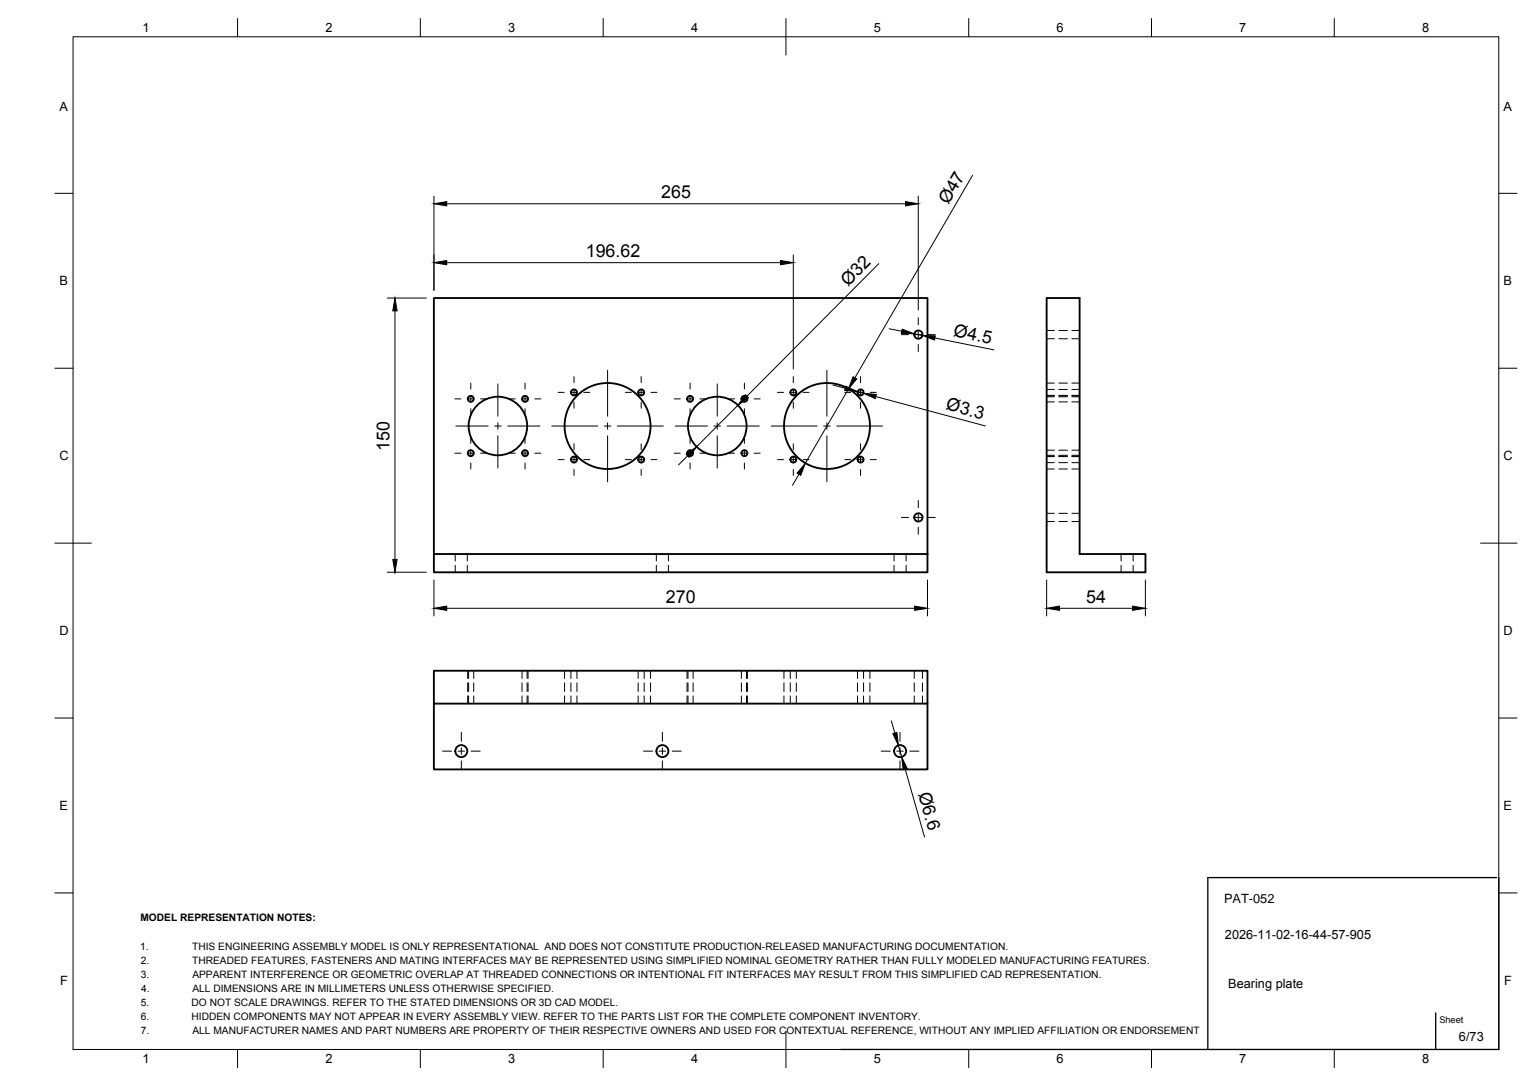
ISO-10303-21;
HEADER;
/* Generated by software containing ST-Developer
 * from STEP Tools, Inc. (www.steptools.com) 
 */

FILE_DESCRIPTION(
/* description */ ('Hand-crank gear train demonstrator'),
/* implementation_level */ '2;1');

FILE_NAME(
/* name */ 'Bearing plate.step',
/* time_stamp */ '2026-10-28T03:22:13-07:00',
/* author */ (''),
/* organization */ (''),
/* preprocessor_version */ 'ST-DEVELOPER v20.2',
/* originating_system */ 'Autodesk Translation Framework v15.17.0.0',
/* authorisation */ '');

FILE_SCHEMA (('AUTOMOTIVE_DESIGN { 1 0 10303 214 3 1 1 }'));
ENDSEC;

DATA;
#10=MECHANICAL_DESIGN_GEOMETRIC_PRESENTATION_REPRESENTATION('',(#1190),#62758);
#1062=SHAPE_REPRESENTATION_RELATIONSHIP('SRR','None',#63034,#1126);
#1126=ADVANCED_BREP_SHAPE_REPRESENTATION('',(#1269),#62688);
#1190=STYLED_ITEM('',(#63462),#1269);
#1269=MANIFOLD_SOLID_BREP('Body1',#16370);
#1348=FACE_BOUND('',#3100,.T.);
#1349=FACE_BOUND('',#3101,.T.);
#1350=FACE_BOUND('',#3102,.T.);
#1351=FACE_BOUND('',#3105,.T.);
#1352=FACE_BOUND('',#3106,.T.);
#1353=FACE_BOUND('',#3107,.T.);
#1354=FACE_BOUND('',#3108,.T.);
#1355=FACE_BOUND('',#3109,.T.);
#1356=FACE_BOUND('',#3110,.T.);
#1357=FACE_BOUND('',#3111,.T.);
#1358=FACE_BOUND('',#3112,.T.);
#1359=FACE_BOUND('',#3113,.T.);
#1360=FACE_BOUND('',#3114,.T.);
#1361=FACE_BOUND('',#3115,.T.);
#1362=FACE_BOUND('',#3116,.T.);
#1363=FACE_BOUND('',#3117,.T.);
#1364=FACE_BOUND('',#3118,.T.);
#1365=FACE_BOUND('',#3119,.T.);
#1366=FACE_BOUND('',#3120,.T.);
#1367=FACE_BOUND('',#3121,.T.);
#1368=FACE_BOUND('',#3122,.T.);
#1369=FACE_BOUND('',#3123,.T.);
#1370=FACE_BOUND('',#3124,.T.);
#1371=FACE_BOUND('',#3125,.T.);
#1372=FACE_BOUND('',#3126,.T.);
#1373=FACE_BOUND('',#3129,.T.);
#1374=FACE_BOUND('',#3130,.T.);
#1375=FACE_BOUND('',#3131,.T.);
#1376=FACE_BOUND('',#3132,.T.);
#1377=FACE_BOUND('',#3133,.T.);
#1378=FACE_BOUND('',#3134,.T.);
#1379=FACE_BOUND('',#3135,.T.);
#1380=FACE_BOUND('',#3136,.T.);
#1381=FACE_BOUND('',#3137,.T.);
#1382=FACE_BOUND('',#3138,.T.);
#1383=FACE_BOUND('',#3139,.T.);
#1384=FACE_BOUND('',#3140,.T.);
#1385=FACE_BOUND('',#3141,.T.);
#1386=FACE_BOUND('',#3142,.T.);
#1387=FACE_BOUND('',#3143,.T.);
#1388=FACE_BOUND('',#3144,.T.);
#1389=FACE_BOUND('',#3145,.T.);
#1390=FACE_BOUND('',#3146,.T.);
#1391=FACE_BOUND('',#3147,.T.);
#1392=FACE_BOUND('',#3148,.T.);
#1393=FACE_BOUND('',#3149,.T.);
#1394=FACE_BOUND('',#3150,.T.);
#1395=FACE_BOUND('',#3154,.T.);
#1396=FACE_BOUND('',#3155,.T.);
#1397=FACE_BOUND('',#3156,.T.);
#1639=PLANE('',#17252);
#1640=PLANE('',#17253);
#1641=PLANE('',#17254);
#1642=PLANE('',#17255);
#1643=PLANE('',#17256);
#1644=PLANE('',#17257);
#1645=PLANE('',#17258);
#1646=PLANE('',#17259);
#2132=FACE_OUTER_BOUND('',#3074,.T.);
#2133=FACE_OUTER_BOUND('',#3075,.T.);
#2134=FACE_OUTER_BOUND('',#3076,.T.);
#2135=FACE_OUTER_BOUND('',#3077,.T.);
#2136=FACE_OUTER_BOUND('',#3078,.T.);
#2137=FACE_OUTER_BOUND('',#3079,.T.);
#2138=FACE_OUTER_BOUND('',#3080,.T.);
#2139=FACE_OUTER_BOUND('',#3081,.T.);
#2140=FACE_OUTER_BOUND('',#3082,.T.);
#2141=FACE_OUTER_BOUND('',#3083,.T.);
#2142=FACE_OUTER_BOUND('',#3084,.T.);
#2143=FACE_OUTER_BOUND('',#3085,.T.);
#2144=FACE_OUTER_BOUND('',#3086,.T.);
#2145=FACE_OUTER_BOUND('',#3087,.T.);
#2146=FACE_OUTER_BOUND('',#3088,.T.);
#2147=FACE_OUTER_BOUND('',#3089,.T.);
#2148=FACE_OUTER_BOUND('',#3090,.T.);
#2149=FACE_OUTER_BOUND('',#3091,.T.);
#2150=FACE_OUTER_BOUND('',#3092,.T.);
#2151=FACE_OUTER_BOUND('',#3093,.T.);
#2152=FACE_OUTER_BOUND('',#3094,.T.);
#2153=FACE_OUTER_BOUND('',#3095,.T.);
#2154=FACE_OUTER_BOUND('',#3096,.T.);
#2155=FACE_OUTER_BOUND('',#3097,.T.);
#2156=FACE_OUTER_BOUND('',#3098,.T.);
#2157=FACE_OUTER_BOUND('',#3099,.T.);
#2158=FACE_OUTER_BOUND('',#3103,.T.);
#2159=FACE_OUTER_BOUND('',#3104,.T.);
#2160=FACE_OUTER_BOUND('',#3127,.T.);
#2161=FACE_OUTER_BOUND('',#3128,.T.);
#2162=FACE_OUTER_BOUND('',#3151,.T.);
#2163=FACE_OUTER_BOUND('',#3152,.T.);
#2164=FACE_OUTER_BOUND('',#3153,.T.);
#3074=EDGE_LOOP('',(#10877,#10878,#10879,#10880));
#3075=EDGE_LOOP('',(#10881,#10882,#10883,#10884));
#3076=EDGE_LOOP('',(#10885,#10886,#10887,#10888));
#3077=EDGE_LOOP('',(#10889,#10890,#10891,#10892));
#3078=EDGE_LOOP('',(#10893,#10894,#10895,#10896));
#3079=EDGE_LOOP('',(#10897,#10898,#10899,#10900));
#3080=EDGE_LOOP('',(#10901,#10902,#10903,#10904));
#3081=EDGE_LOOP('',(#10905,#10906,#10907,#10908));
#3082=EDGE_LOOP('',(#10909,#10910,#10911,#10912));
#3083=EDGE_LOOP('',(#10913,#10914,#10915,#10916));
#3084=EDGE_LOOP('',(#10917,#10918,#10919,#10920));
#3085=EDGE_LOOP('',(#10921,#10922,#10923,#10924));
#3086=EDGE_LOOP('',(#10925,#10926,#10927,#10928));
#3087=EDGE_LOOP('',(#10929,#10930,#10931,#10932));
#3088=EDGE_LOOP('',(#10933,#10934,#10935,#10936));
#3089=EDGE_LOOP('',(#10937,#10938,#10939,#10940));
#3090=EDGE_LOOP('',(#10941,#10942,#10943,#10944));
#3091=EDGE_LOOP('',(#10945,#10946,#10947,#10948));
#3092=EDGE_LOOP('',(#10949,#10950,#10951,#10952));
#3093=EDGE_LOOP('',(#10953,#10954,#10955,#10956));
#3094=EDGE_LOOP('',(#10957,#10958,#10959,#10960));
#3095=EDGE_LOOP('',(#10961,#10962,#10963,#10964));
#3096=EDGE_LOOP('',(#10965,#10966,#10967,#10968));
#3097=EDGE_LOOP('',(#10969,#10970,#10971,#10972));
#3098=EDGE_LOOP('',(#10973,#10974,#10975,#10976));
#3099=EDGE_LOOP('',(#10977,#10978,#10979,#10980));
#3100=EDGE_LOOP('',(#10981));
#3101=EDGE_LOOP('',(#10982));
#3102=EDGE_LOOP('',(#10983));
#3103=EDGE_LOOP('',(#10984,#10985,#10986,#10987));
#3104=EDGE_LOOP('',(#10988,#10989,#10990,#10991));
#3105=EDGE_LOOP('',(#10992));
#3106=EDGE_LOOP('',(#10993));
#3107=EDGE_LOOP('',(#10994));
#3108=EDGE_LOOP('',(#10995));
#3109=EDGE_LOOP('',(#10996));
#3110=EDGE_LOOP('',(#10997));
#3111=EDGE_LOOP('',(#10998));
#3112=EDGE_LOOP('',(#10999));
#3113=EDGE_LOOP('',(#11000));
#3114=EDGE_LOOP('',(#11001));
#3115=EDGE_LOOP('',(#11002));
#3116=EDGE_LOOP('',(#11003));
#3117=EDGE_LOOP('',(#11004));
#3118=EDGE_LOOP('',(#11005));
#3119=EDGE_LOOP('',(#11006));
#3120=EDGE_LOOP('',(#11007));
#3121=EDGE_LOOP('',(#11008));
#3122=EDGE_LOOP('',(#11009));
#3123=EDGE_LOOP('',(#11010));
#3124=EDGE_LOOP('',(#11011));
#3125=EDGE_LOOP('',(#11012));
#3126=EDGE_LOOP('',(#11013));
#3127=EDGE_LOOP('',(#11014,#11015,#11016,#11017,#11018,#11019));
#3128=EDGE_LOOP('',(#11020,#11021,#11022,#11023));
#3129=EDGE_LOOP('',(#11024));
#3130=EDGE_LOOP('',(#11025));
#3131=EDGE_LOOP('',(#11026));
#3132=EDGE_LOOP('',(#11027));
#3133=EDGE_LOOP('',(#11028));
#3134=EDGE_LOOP('',(#11029));
#3135=EDGE_LOOP('',(#11030));
#3136=EDGE_LOOP('',(#11031));
#3137=EDGE_LOOP('',(#11032));
#3138=EDGE_LOOP('',(#11033));
#3139=EDGE_LOOP('',(#11034));
#3140=EDGE_LOOP('',(#11035));
#3141=EDGE_LOOP('',(#11036));
#3142=EDGE_LOOP('',(#11037));
#3143=EDGE_LOOP('',(#11038));
#3144=EDGE_LOOP('',(#11039));
#3145=EDGE_LOOP('',(#11040));
#3146=EDGE_LOOP('',(#11041));
#3147=EDGE_LOOP('',(#11042));
#3148=EDGE_LOOP('',(#11043));
#3149=EDGE_LOOP('',(#11044));
#3150=EDGE_LOOP('',(#11045));
#3151=EDGE_LOOP('',(#11046,#11047,#11048,#11049,#11050,#11051));
#3152=EDGE_LOOP('',(#11052,#11053,#11054,#11055));
#3153=EDGE_LOOP('',(#11056,#11057,#11058,#11059));
#3154=EDGE_LOOP('',(#11060));
#3155=EDGE_LOOP('',(#11061));
#3156=EDGE_LOOP('',(#11062));
#4301=LINE('',#23361,#5433);
#4302=LINE('',#23367,#5434);
#4303=LINE('',#23373,#5435);
#4304=LINE('',#23379,#5436);
#4305=LINE('',#23385,#5437);
#4306=LINE('',#23391,#5438);
#4307=LINE('',#23397,#5439);
#4308=LINE('',#23403,#5440);
#4309=LINE('',#23409,#5441);
#4310=LINE('',#23415,#5442);
#4311=LINE('',#23421,#5443);
#4312=LINE('',#23427,#5444);
#4313=LINE('',#23433,#5445);
#4314=LINE('',#23439,#5446);
#4315=LINE('',#23445,#5447);
#4316=LINE('',#23451,#5448);
#4317=LINE('',#23457,#5449);
#4318=LINE('',#23463,#5450);
#4319=LINE('',#23469,#5451);
#4320=LINE('',#23475,#5452);
#4321=LINE('',#23481,#5453);
#4322=LINE('',#23487,#5454);
#4323=LINE('',#23493,#5455);
#4324=LINE('',#23499,#5456);
#4325=LINE('',#23505,#5457);
#4326=LINE('',#23510,#5458);
#4327=LINE('',#23512,#5459);
#4328=LINE('',#23514,#5460);
#4329=LINE('',#23515,#5461);
#4330=LINE('',#23518,#5462);
#4331=LINE('',#23520,#5463);
#4332=LINE('',#23521,#5464);
#4333=LINE('',#23525,#5465);
#4334=LINE('',#23527,#5466);
#4335=LINE('',#23529,#5467);
#4336=LINE('',#23530,#5468);
#4337=LINE('',#23532,#5469);
#4338=LINE('',#23534,#5470);
#4339=LINE('',#23535,#5471);
#4340=LINE('',#23538,#5472);
#4341=LINE('',#23539,#5473);
#4342=LINE('',#23541,#5474);
#4343=LINE('',#23542,#5475);
#5433=VECTOR('',#18888,0.225000000000001);
#5434=VECTOR('',#18895,0.225000000000001);
#5435=VECTOR('',#18902,0.164999999999999);
#5436=VECTOR('',#18909,0.164999999999999);
#5437=VECTOR('',#18916,0.164999999999999);
#5438=VECTOR('',#18923,0.164999999999999);
#5439=VECTOR('',#18930,2.35);
#5440=VECTOR('',#18937,0.164999999999999);
#5441=VECTOR('',#18944,0.164999999999999);
#5442=VECTOR('',#18951,0.164999999999999);
#5443=VECTOR('',#18958,0.164999999999999);
#5444=VECTOR('',#18965,1.6);
#5445=VECTOR('',#18972,0.165);
#5446=VECTOR('',#18979,0.165);
#5447=VECTOR('',#18986,0.165);
#5448=VECTOR('',#18993,0.165);
#5449=VECTOR('',#19000,2.35);
#5450=VECTOR('',#19007,0.165);
#5451=VECTOR('',#19014,0.165);
#5452=VECTOR('',#19021,0.165);
#5453=VECTOR('',#19028,0.165);
#5454=VECTOR('',#19035,1.6);
#5455=VECTOR('',#19042,0.33);
#5456=VECTOR('',#19049,0.33);
#5457=VECTOR('',#19056,0.329999999999998);
#5458=VECTOR('',#19061,1.);
#5459=VECTOR('',#19062,1.);
#5460=VECTOR('',#19063,1.);
#5461=VECTOR('',#19064,1.);
#5462=VECTOR('',#19067,1.);
#5463=VECTOR('',#19068,1.);
#5464=VECTOR('',#19069,1.);
#5465=VECTOR('',#19072,1.);
#5466=VECTOR('',#19073,1.);
#5467=VECTOR('',#19074,1.);
#5468=VECTOR('',#19075,1.);
#5469=VECTOR('',#19078,1.);
#5470=VECTOR('',#19079,1.);
#5471=VECTOR('',#19080,1.);
#5472=VECTOR('',#19083,1.);
#5473=VECTOR('',#19084,1.);
#5474=VECTOR('',#19087,1.);
#5475=VECTOR('',#19088,1.);
#6556=CIRCLE('',#17178,0.225000000000001);
#6557=CIRCLE('',#17179,0.225000000000001);
#6558=CIRCLE('',#17181,0.225000000000001);
#6559=CIRCLE('',#17182,0.225000000000001);
#6560=CIRCLE('',#17184,0.164999999999999);
#6561=CIRCLE('',#17185,0.164999999999999);
#6562=CIRCLE('',#17187,0.164999999999999);
#6563=CIRCLE('',#17188,0.164999999999999);
#6564=CIRCLE('',#17190,0.164999999999999);
#6565=CIRCLE('',#17191,0.164999999999999);
#6566=CIRCLE('',#17193,0.164999999999999);
#6567=CIRCLE('',#17194,0.164999999999999);
#6568=CIRCLE('',#17196,2.35);
#6569=CIRCLE('',#17197,2.35);
#6570=CIRCLE('',#17199,0.164999999999999);
#6571=CIRCLE('',#17200,0.164999999999999);
#6572=CIRCLE('',#17202,0.164999999999999);
#6573=CIRCLE('',#17203,0.164999999999999);
#6574=CIRCLE('',#17205,0.164999999999999);
#6575=CIRCLE('',#17206,0.164999999999999);
#6576=CIRCLE('',#17208,0.164999999999999);
#6577=CIRCLE('',#17209,0.164999999999999);
#6578=CIRCLE('',#17211,1.6);
#6579=CIRCLE('',#17212,1.6);
#6580=CIRCLE('',#17214,0.165);
#6581=CIRCLE('',#17215,0.165);
#6582=CIRCLE('',#17217,0.165);
#6583=CIRCLE('',#17218,0.165);
#6584=CIRCLE('',#17220,0.165);
#6585=CIRCLE('',#17221,0.165);
#6586=CIRCLE('',#17223,0.165);
#6587=CIRCLE('',#17224,0.165);
#6588=CIRCLE('',#17226,2.35);
#6589=CIRCLE('',#17227,2.35);
#6590=CIRCLE('',#17229,0.165);
#6591=CIRCLE('',#17230,0.165);
#6592=CIRCLE('',#17232,0.165);
#6593=CIRCLE('',#17233,0.165);
#6594=CIRCLE('',#17235,0.165);
#6595=CIRCLE('',#17236,0.165);
#6596=CIRCLE('',#17238,0.165);
#6597=CIRCLE('',#17239,0.165);
#6598=CIRCLE('',#17241,1.6);
#6599=CIRCLE('',#17242,1.6);
#6600=CIRCLE('',#17244,0.33);
#6601=CIRCLE('',#17245,0.33);
#6602=CIRCLE('',#17247,0.33);
#6603=CIRCLE('',#17248,0.33);
#6604=CIRCLE('',#17250,0.329999999999998);
#6605=CIRCLE('',#17251,0.329999999999998);
#7226=VERTEX_POINT('',#23358);
#7227=VERTEX_POINT('',#23360);
#7228=VERTEX_POINT('',#23364);
#7229=VERTEX_POINT('',#23366);
#7230=VERTEX_POINT('',#23370);
#7231=VERTEX_POINT('',#23372);
#7232=VERTEX_POINT('',#23376);
#7233=VERTEX_POINT('',#23378);
#7234=VERTEX_POINT('',#23382);
#7235=VERTEX_POINT('',#23384);
#7236=VERTEX_POINT('',#23388);
#7237=VERTEX_POINT('',#23390);
#7238=VERTEX_POINT('',#23394);
#7239=VERTEX_POINT('',#23396);
#7240=VERTEX_POINT('',#23400);
#7241=VERTEX_POINT('',#23402);
#7242=VERTEX_POINT('',#23406);
#7243=VERTEX_POINT('',#23408);
#7244=VERTEX_POINT('',#23412);
#7245=VERTEX_POINT('',#23414);
#7246=VERTEX_POINT('',#23418);
#7247=VERTEX_POINT('',#23420);
#7248=VERTEX_POINT('',#23424);
#7249=VERTEX_POINT('',#23426);
#7250=VERTEX_POINT('',#23430);
#7251=VERTEX_POINT('',#23432);
#7252=VERTEX_POINT('',#23436);
#7253=VERTEX_POINT('',#23438);
#7254=VERTEX_POINT('',#23442);
#7255=VERTEX_POINT('',#23444);
#7256=VERTEX_POINT('',#23448);
#7257=VERTEX_POINT('',#23450);
#7258=VERTEX_POINT('',#23454);
#7259=VERTEX_POINT('',#23456);
#7260=VERTEX_POINT('',#23460);
#7261=VERTEX_POINT('',#23462);
#7262=VERTEX_POINT('',#23466);
#7263=VERTEX_POINT('',#23468);
#7264=VERTEX_POINT('',#23472);
#7265=VERTEX_POINT('',#23474);
#7266=VERTEX_POINT('',#23478);
#7267=VERTEX_POINT('',#23480);
#7268=VERTEX_POINT('',#23484);
#7269=VERTEX_POINT('',#23486);
#7270=VERTEX_POINT('',#23490);
#7271=VERTEX_POINT('',#23492);
#7272=VERTEX_POINT('',#23496);
#7273=VERTEX_POINT('',#23498);
#7274=VERTEX_POINT('',#23502);
#7275=VERTEX_POINT('',#23504);
#7276=VERTEX_POINT('',#23508);
#7277=VERTEX_POINT('',#23509);
#7278=VERTEX_POINT('',#23511);
#7279=VERTEX_POINT('',#23513);
#7280=VERTEX_POINT('',#23517);
#7281=VERTEX_POINT('',#23519);
#7282=VERTEX_POINT('',#23523);
#7283=VERTEX_POINT('',#23524);
#7284=VERTEX_POINT('',#23526);
#7285=VERTEX_POINT('',#23528);
#7286=VERTEX_POINT('',#23533);
#7287=VERTEX_POINT('',#23537);
#8690=EDGE_CURVE('',#7226,#7226,#6556,.T.);
#8691=EDGE_CURVE('',#7226,#7227,#4301,.T.);
#8692=EDGE_CURVE('',#7227,#7227,#6557,.T.);
#8693=EDGE_CURVE('',#7228,#7228,#6558,.T.);
#8694=EDGE_CURVE('',#7228,#7229,#4302,.T.);
#8695=EDGE_CURVE('',#7229,#7229,#6559,.T.);
#8696=EDGE_CURVE('',#7230,#7230,#6560,.T.);
#8697=EDGE_CURVE('',#7230,#7231,#4303,.T.);
#8698=EDGE_CURVE('',#7231,#7231,#6561,.T.);
#8699=EDGE_CURVE('',#7232,#7232,#6562,.T.);
#8700=EDGE_CURVE('',#7232,#7233,#4304,.T.);
#8701=EDGE_CURVE('',#7233,#7233,#6563,.T.);
#8702=EDGE_CURVE('',#7234,#7234,#6564,.T.);
#8703=EDGE_CURVE('',#7234,#7235,#4305,.T.);
#8704=EDGE_CURVE('',#7235,#7235,#6565,.T.);
#8705=EDGE_CURVE('',#7236,#7236,#6566,.T.);
#8706=EDGE_CURVE('',#7236,#7237,#4306,.T.);
#8707=EDGE_CURVE('',#7237,#7237,#6567,.T.);
#8708=EDGE_CURVE('',#7238,#7238,#6568,.T.);
#8709=EDGE_CURVE('',#7238,#7239,#4307,.T.);
#8710=EDGE_CURVE('',#7239,#7239,#6569,.T.);
#8711=EDGE_CURVE('',#7240,#7240,#6570,.T.);
#8712=EDGE_CURVE('',#7240,#7241,#4308,.T.);
#8713=EDGE_CURVE('',#7241,#7241,#6571,.T.);
#8714=EDGE_CURVE('',#7242,#7242,#6572,.T.);
#8715=EDGE_CURVE('',#7242,#7243,#4309,.T.);
#8716=EDGE_CURVE('',#7243,#7243,#6573,.T.);
#8717=EDGE_CURVE('',#7244,#7244,#6574,.T.);
#8718=EDGE_CURVE('',#7244,#7245,#4310,.T.);
#8719=EDGE_CURVE('',#7245,#7245,#6575,.T.);
#8720=EDGE_CURVE('',#7246,#7246,#6576,.T.);
#8721=EDGE_CURVE('',#7246,#7247,#4311,.T.);
#8722=EDGE_CURVE('',#7247,#7247,#6577,.T.);
#8723=EDGE_CURVE('',#7248,#7248,#6578,.T.);
#8724=EDGE_CURVE('',#7248,#7249,#4312,.T.);
#8725=EDGE_CURVE('',#7249,#7249,#6579,.T.);
#8726=EDGE_CURVE('',#7250,#7250,#6580,.T.);
#8727=EDGE_CURVE('',#7250,#7251,#4313,.T.);
#8728=EDGE_CURVE('',#7251,#7251,#6581,.T.);
#8729=EDGE_CURVE('',#7252,#7252,#6582,.T.);
#8730=EDGE_CURVE('',#7252,#7253,#4314,.T.);
#8731=EDGE_CURVE('',#7253,#7253,#6583,.T.);
#8732=EDGE_CURVE('',#7254,#7254,#6584,.T.);
#8733=EDGE_CURVE('',#7254,#7255,#4315,.T.);
#8734=EDGE_CURVE('',#7255,#7255,#6585,.T.);
#8735=EDGE_CURVE('',#7256,#7256,#6586,.T.);
#8736=EDGE_CURVE('',#7256,#7257,#4316,.T.);
#8737=EDGE_CURVE('',#7257,#7257,#6587,.T.);
#8738=EDGE_CURVE('',#7258,#7258,#6588,.T.);
#8739=EDGE_CURVE('',#7258,#7259,#4317,.T.);
#8740=EDGE_CURVE('',#7259,#7259,#6589,.T.);
#8741=EDGE_CURVE('',#7260,#7260,#6590,.T.);
#8742=EDGE_CURVE('',#7260,#7261,#4318,.T.);
#8743=EDGE_CURVE('',#7261,#7261,#6591,.T.);
#8744=EDGE_CURVE('',#7262,#7262,#6592,.T.);
#8745=EDGE_CURVE('',#7262,#7263,#4319,.T.);
#8746=EDGE_CURVE('',#7263,#7263,#6593,.T.);
#8747=EDGE_CURVE('',#7264,#7264,#6594,.T.);
#8748=EDGE_CURVE('',#7264,#7265,#4320,.T.);
#8749=EDGE_CURVE('',#7265,#7265,#6595,.T.);
#8750=EDGE_CURVE('',#7266,#7266,#6596,.T.);
#8751=EDGE_CURVE('',#7266,#7267,#4321,.T.);
#8752=EDGE_CURVE('',#7267,#7267,#6597,.T.);
#8753=EDGE_CURVE('',#7268,#7268,#6598,.T.);
#8754=EDGE_CURVE('',#7268,#7269,#4322,.T.);
#8755=EDGE_CURVE('',#7269,#7269,#6599,.T.);
#8756=EDGE_CURVE('',#7270,#7270,#6600,.T.);
#8757=EDGE_CURVE('',#7270,#7271,#4323,.T.);
#8758=EDGE_CURVE('',#7271,#7271,#6601,.T.);
#8759=EDGE_CURVE('',#7272,#7272,#6602,.T.);
#8760=EDGE_CURVE('',#7272,#7273,#4324,.T.);
#8761=EDGE_CURVE('',#7273,#7273,#6603,.T.);
#8762=EDGE_CURVE('',#7274,#7274,#6604,.T.);
#8763=EDGE_CURVE('',#7274,#7275,#4325,.T.);
#8764=EDGE_CURVE('',#7275,#7275,#6605,.T.);
#8765=EDGE_CURVE('',#7276,#7277,#4326,.T.);
#8766=EDGE_CURVE('',#7276,#7278,#4327,.T.);
#8767=EDGE_CURVE('',#7279,#7278,#4328,.T.);
#8768=EDGE_CURVE('',#7277,#7279,#4329,.T.);
#8769=EDGE_CURVE('',#7277,#7280,#4330,.T.);
#8770=EDGE_CURVE('',#7280,#7281,#4331,.T.);
#8771=EDGE_CURVE('',#7281,#7276,#4332,.T.);
#8772=EDGE_CURVE('',#7282,#7283,#4333,.T.);
#8773=EDGE_CURVE('',#7283,#7284,#4334,.T.);
#8774=EDGE_CURVE('',#7285,#7284,#4335,.T.);
#8775=EDGE_CURVE('',#7282,#7285,#4336,.T.);
#8776=EDGE_CURVE('',#7281,#7282,#4337,.T.);
#8777=EDGE_CURVE('',#7286,#7285,#4338,.T.);
#8778=EDGE_CURVE('',#7278,#7286,#4339,.T.);
#8779=EDGE_CURVE('',#7287,#7286,#4340,.T.);
#8780=EDGE_CURVE('',#7279,#7287,#4341,.T.);
#8781=EDGE_CURVE('',#7283,#7280,#4342,.T.);
#8782=EDGE_CURVE('',#7284,#7287,#4343,.T.);
#10877=ORIENTED_EDGE('',*,*,#8690,.F.);
#10878=ORIENTED_EDGE('',*,*,#8691,.T.);
#10879=ORIENTED_EDGE('',*,*,#8692,.F.);
#10880=ORIENTED_EDGE('',*,*,#8691,.F.);
#10881=ORIENTED_EDGE('',*,*,#8693,.F.);
#10882=ORIENTED_EDGE('',*,*,#8694,.T.);
#10883=ORIENTED_EDGE('',*,*,#8695,.F.);
#10884=ORIENTED_EDGE('',*,*,#8694,.F.);
#10885=ORIENTED_EDGE('',*,*,#8696,.F.);
#10886=ORIENTED_EDGE('',*,*,#8697,.T.);
#10887=ORIENTED_EDGE('',*,*,#8698,.F.);
#10888=ORIENTED_EDGE('',*,*,#8697,.F.);
#10889=ORIENTED_EDGE('',*,*,#8699,.F.);
#10890=ORIENTED_EDGE('',*,*,#8700,.T.);
#10891=ORIENTED_EDGE('',*,*,#8701,.F.);
#10892=ORIENTED_EDGE('',*,*,#8700,.F.);
#10893=ORIENTED_EDGE('',*,*,#8702,.F.);
#10894=ORIENTED_EDGE('',*,*,#8703,.T.);
#10895=ORIENTED_EDGE('',*,*,#8704,.F.);
#10896=ORIENTED_EDGE('',*,*,#8703,.F.);
#10897=ORIENTED_EDGE('',*,*,#8705,.F.);
#10898=ORIENTED_EDGE('',*,*,#8706,.T.);
#10899=ORIENTED_EDGE('',*,*,#8707,.F.);
#10900=ORIENTED_EDGE('',*,*,#8706,.F.);
#10901=ORIENTED_EDGE('',*,*,#8708,.F.);
#10902=ORIENTED_EDGE('',*,*,#8709,.T.);
#10903=ORIENTED_EDGE('',*,*,#8710,.F.);
#10904=ORIENTED_EDGE('',*,*,#8709,.F.);
#10905=ORIENTED_EDGE('',*,*,#8711,.F.);
#10906=ORIENTED_EDGE('',*,*,#8712,.T.);
#10907=ORIENTED_EDGE('',*,*,#8713,.F.);
#10908=ORIENTED_EDGE('',*,*,#8712,.F.);
#10909=ORIENTED_EDGE('',*,*,#8714,.F.);
#10910=ORIENTED_EDGE('',*,*,#8715,.T.);
#10911=ORIENTED_EDGE('',*,*,#8716,.F.);
#10912=ORIENTED_EDGE('',*,*,#8715,.F.);
#10913=ORIENTED_EDGE('',*,*,#8717,.F.);
#10914=ORIENTED_EDGE('',*,*,#8718,.T.);
#10915=ORIENTED_EDGE('',*,*,#8719,.F.);
#10916=ORIENTED_EDGE('',*,*,#8718,.F.);
#10917=ORIENTED_EDGE('',*,*,#8720,.F.);
#10918=ORIENTED_EDGE('',*,*,#8721,.T.);
#10919=ORIENTED_EDGE('',*,*,#8722,.F.);
#10920=ORIENTED_EDGE('',*,*,#8721,.F.);
#10921=ORIENTED_EDGE('',*,*,#8723,.F.);
#10922=ORIENTED_EDGE('',*,*,#8724,.T.);
#10923=ORIENTED_EDGE('',*,*,#8725,.F.);
#10924=ORIENTED_EDGE('',*,*,#8724,.F.);
#10925=ORIENTED_EDGE('',*,*,#8726,.F.);
#10926=ORIENTED_EDGE('',*,*,#8727,.T.);
#10927=ORIENTED_EDGE('',*,*,#8728,.F.);
#10928=ORIENTED_EDGE('',*,*,#8727,.F.);
#10929=ORIENTED_EDGE('',*,*,#8729,.F.);
#10930=ORIENTED_EDGE('',*,*,#8730,.T.);
#10931=ORIENTED_EDGE('',*,*,#8731,.F.);
#10932=ORIENTED_EDGE('',*,*,#8730,.F.);
#10933=ORIENTED_EDGE('',*,*,#8732,.F.);
#10934=ORIENTED_EDGE('',*,*,#8733,.T.);
#10935=ORIENTED_EDGE('',*,*,#8734,.F.);
#10936=ORIENTED_EDGE('',*,*,#8733,.F.);
#10937=ORIENTED_EDGE('',*,*,#8735,.F.);
#10938=ORIENTED_EDGE('',*,*,#8736,.T.);
#10939=ORIENTED_EDGE('',*,*,#8737,.F.);
#10940=ORIENTED_EDGE('',*,*,#8736,.F.);
#10941=ORIENTED_EDGE('',*,*,#8738,.F.);
#10942=ORIENTED_EDGE('',*,*,#8739,.T.);
#10943=ORIENTED_EDGE('',*,*,#8740,.F.);
#10944=ORIENTED_EDGE('',*,*,#8739,.F.);
#10945=ORIENTED_EDGE('',*,*,#8741,.F.);
#10946=ORIENTED_EDGE('',*,*,#8742,.T.);
#10947=ORIENTED_EDGE('',*,*,#8743,.F.);
#10948=ORIENTED_EDGE('',*,*,#8742,.F.);
#10949=ORIENTED_EDGE('',*,*,#8744,.F.);
#10950=ORIENTED_EDGE('',*,*,#8745,.T.);
#10951=ORIENTED_EDGE('',*,*,#8746,.F.);
#10952=ORIENTED_EDGE('',*,*,#8745,.F.);
#10953=ORIENTED_EDGE('',*,*,#8747,.F.);
#10954=ORIENTED_EDGE('',*,*,#8748,.T.);
#10955=ORIENTED_EDGE('',*,*,#8749,.F.);
#10956=ORIENTED_EDGE('',*,*,#8748,.F.);
#10957=ORIENTED_EDGE('',*,*,#8750,.F.);
#10958=ORIENTED_EDGE('',*,*,#8751,.T.);
#10959=ORIENTED_EDGE('',*,*,#8752,.F.);
#10960=ORIENTED_EDGE('',*,*,#8751,.F.);
#10961=ORIENTED_EDGE('',*,*,#8753,.F.);
#10962=ORIENTED_EDGE('',*,*,#8754,.T.);
#10963=ORIENTED_EDGE('',*,*,#8755,.F.);
#10964=ORIENTED_EDGE('',*,*,#8754,.F.);
#10965=ORIENTED_EDGE('',*,*,#8756,.F.);
#10966=ORIENTED_EDGE('',*,*,#8757,.T.);
#10967=ORIENTED_EDGE('',*,*,#8758,.F.);
#10968=ORIENTED_EDGE('',*,*,#8757,.F.);
#10969=ORIENTED_EDGE('',*,*,#8759,.F.);
#10970=ORIENTED_EDGE('',*,*,#8760,.T.);
#10971=ORIENTED_EDGE('',*,*,#8761,.F.);
#10972=ORIENTED_EDGE('',*,*,#8760,.F.);
#10973=ORIENTED_EDGE('',*,*,#8762,.F.);
#10974=ORIENTED_EDGE('',*,*,#8763,.T.);
#10975=ORIENTED_EDGE('',*,*,#8764,.F.);
#10976=ORIENTED_EDGE('',*,*,#8763,.F.);
#10977=ORIENTED_EDGE('',*,*,#8765,.F.);
#10978=ORIENTED_EDGE('',*,*,#8766,.T.);
#10979=ORIENTED_EDGE('',*,*,#8767,.F.);
#10980=ORIENTED_EDGE('',*,*,#8768,.F.);
#10981=ORIENTED_EDGE('',*,*,#8758,.T.);
#10982=ORIENTED_EDGE('',*,*,#8761,.T.);
#10983=ORIENTED_EDGE('',*,*,#8764,.T.);
#10984=ORIENTED_EDGE('',*,*,#8765,.T.);
#10985=ORIENTED_EDGE('',*,*,#8769,.T.);
#10986=ORIENTED_EDGE('',*,*,#8770,.T.);
#10987=ORIENTED_EDGE('',*,*,#8771,.T.);
#10988=ORIENTED_EDGE('',*,*,#8772,.T.);
#10989=ORIENTED_EDGE('',*,*,#8773,.T.);
#10990=ORIENTED_EDGE('',*,*,#8774,.F.);
#10991=ORIENTED_EDGE('',*,*,#8775,.F.);
#10992=ORIENTED_EDGE('',*,*,#8695,.T.);
#10993=ORIENTED_EDGE('',*,*,#8710,.T.);
#10994=ORIENTED_EDGE('',*,*,#8725,.T.);
#10995=ORIENTED_EDGE('',*,*,#8743,.T.);
#10996=ORIENTED_EDGE('',*,*,#8746,.T.);
#10997=ORIENTED_EDGE('',*,*,#8749,.T.);
#10998=ORIENTED_EDGE('',*,*,#8752,.T.);
#10999=ORIENTED_EDGE('',*,*,#8755,.T.);
#11000=ORIENTED_EDGE('',*,*,#8740,.T.);
#11001=ORIENTED_EDGE('',*,*,#8737,.T.);
#11002=ORIENTED_EDGE('',*,*,#8734,.T.);
#11003=ORIENTED_EDGE('',*,*,#8731,.T.);
#11004=ORIENTED_EDGE('',*,*,#8728,.T.);
#11005=ORIENTED_EDGE('',*,*,#8722,.T.);
#11006=ORIENTED_EDGE('',*,*,#8719,.T.);
#11007=ORIENTED_EDGE('',*,*,#8716,.T.);
#11008=ORIENTED_EDGE('',*,*,#8713,.T.);
#11009=ORIENTED_EDGE('',*,*,#8707,.T.);
#11010=ORIENTED_EDGE('',*,*,#8704,.T.);
#11011=ORIENTED_EDGE('',*,*,#8701,.T.);
#11012=ORIENTED_EDGE('',*,*,#8698,.T.);
#11013=ORIENTED_EDGE('',*,*,#8692,.T.);
#11014=ORIENTED_EDGE('',*,*,#8776,.T.);
#11015=ORIENTED_EDGE('',*,*,#8775,.T.);
#11016=ORIENTED_EDGE('',*,*,#8777,.F.);
#11017=ORIENTED_EDGE('',*,*,#8778,.F.);
#11018=ORIENTED_EDGE('',*,*,#8766,.F.);
#11019=ORIENTED_EDGE('',*,*,#8771,.F.);
#11020=ORIENTED_EDGE('',*,*,#8767,.T.);
#11021=ORIENTED_EDGE('',*,*,#8778,.T.);
#11022=ORIENTED_EDGE('',*,*,#8779,.F.);
#11023=ORIENTED_EDGE('',*,*,#8780,.F.);
#11024=ORIENTED_EDGE('',*,*,#8693,.T.);
#11025=ORIENTED_EDGE('',*,*,#8708,.T.);
#11026=ORIENTED_EDGE('',*,*,#8723,.T.);
#11027=ORIENTED_EDGE('',*,*,#8741,.T.);
#11028=ORIENTED_EDGE('',*,*,#8744,.T.);
#11029=ORIENTED_EDGE('',*,*,#8747,.T.);
#11030=ORIENTED_EDGE('',*,*,#8750,.T.);
#11031=ORIENTED_EDGE('',*,*,#8753,.T.);
#11032=ORIENTED_EDGE('',*,*,#8738,.T.);
#11033=ORIENTED_EDGE('',*,*,#8735,.T.);
#11034=ORIENTED_EDGE('',*,*,#8732,.T.);
#11035=ORIENTED_EDGE('',*,*,#8729,.T.);
#11036=ORIENTED_EDGE('',*,*,#8726,.T.);
#11037=ORIENTED_EDGE('',*,*,#8720,.T.);
#11038=ORIENTED_EDGE('',*,*,#8717,.T.);
#11039=ORIENTED_EDGE('',*,*,#8714,.T.);
#11040=ORIENTED_EDGE('',*,*,#8711,.T.);
#11041=ORIENTED_EDGE('',*,*,#8705,.T.);
#11042=ORIENTED_EDGE('',*,*,#8702,.T.);
#11043=ORIENTED_EDGE('',*,*,#8699,.T.);
#11044=ORIENTED_EDGE('',*,*,#8696,.T.);
#11045=ORIENTED_EDGE('',*,*,#8690,.T.);
#11046=ORIENTED_EDGE('',*,*,#8781,.T.);
#11047=ORIENTED_EDGE('',*,*,#8769,.F.);
#11048=ORIENTED_EDGE('',*,*,#8768,.T.);
#11049=ORIENTED_EDGE('',*,*,#8780,.T.);
#11050=ORIENTED_EDGE('',*,*,#8782,.F.);
#11051=ORIENTED_EDGE('',*,*,#8773,.F.);
#11052=ORIENTED_EDGE('',*,*,#8782,.T.);
#11053=ORIENTED_EDGE('',*,*,#8779,.T.);
#11054=ORIENTED_EDGE('',*,*,#8777,.T.);
#11055=ORIENTED_EDGE('',*,*,#8774,.T.);
#11056=ORIENTED_EDGE('',*,*,#8781,.F.);
#11057=ORIENTED_EDGE('',*,*,#8772,.F.);
#11058=ORIENTED_EDGE('',*,*,#8776,.F.);
#11059=ORIENTED_EDGE('',*,*,#8770,.F.);
#11060=ORIENTED_EDGE('',*,*,#8756,.T.);
#11061=ORIENTED_EDGE('',*,*,#8759,.T.);
#11062=ORIENTED_EDGE('',*,*,#8762,.T.);
#15170=CYLINDRICAL_SURFACE('',#17177,0.225000000000001);
#15171=CYLINDRICAL_SURFACE('',#17180,0.225000000000001);
#15172=CYLINDRICAL_SURFACE('',#17183,0.164999999999999);
#15173=CYLINDRICAL_SURFACE('',#17186,0.164999999999999);
#15174=CYLINDRICAL_SURFACE('',#17189,0.164999999999999);
#15175=CYLINDRICAL_SURFACE('',#17192,0.164999999999999);
#15176=CYLINDRICAL_SURFACE('',#17195,2.35);
#15177=CYLINDRICAL_SURFACE('',#17198,0.164999999999999);
#15178=CYLINDRICAL_SURFACE('',#17201,0.164999999999999);
#15179=CYLINDRICAL_SURFACE('',#17204,0.164999999999999);
#15180=CYLINDRICAL_SURFACE('',#17207,0.164999999999999);
#15181=CYLINDRICAL_SURFACE('',#17210,1.6);
#15182=CYLINDRICAL_SURFACE('',#17213,0.165);
#15183=CYLINDRICAL_SURFACE('',#17216,0.165);
#15184=CYLINDRICAL_SURFACE('',#17219,0.165);
#15185=CYLINDRICAL_SURFACE('',#17222,0.165);
#15186=CYLINDRICAL_SURFACE('',#17225,2.35);
#15187=CYLINDRICAL_SURFACE('',#17228,0.165);
#15188=CYLINDRICAL_SURFACE('',#17231,0.165);
#15189=CYLINDRICAL_SURFACE('',#17234,0.165);
#15190=CYLINDRICAL_SURFACE('',#17237,0.165);
#15191=CYLINDRICAL_SURFACE('',#17240,1.6);
#15192=CYLINDRICAL_SURFACE('',#17243,0.33);
#15193=CYLINDRICAL_SURFACE('',#17246,0.33);
#15194=CYLINDRICAL_SURFACE('',#17249,0.329999999999998);
#15442=ADVANCED_FACE('',(#2132),#15170,.F.);
#15443=ADVANCED_FACE('',(#2133),#15171,.F.);
#15444=ADVANCED_FACE('',(#2134),#15172,.F.);
#15445=ADVANCED_FACE('',(#2135),#15173,.F.);
#15446=ADVANCED_FACE('',(#2136),#15174,.F.);
#15447=ADVANCED_FACE('',(#2137),#15175,.F.);
#15448=ADVANCED_FACE('',(#2138),#15176,.F.);
#15449=ADVANCED_FACE('',(#2139),#15177,.F.);
#15450=ADVANCED_FACE('',(#2140),#15178,.F.);
#15451=ADVANCED_FACE('',(#2141),#15179,.F.);
#15452=ADVANCED_FACE('',(#2142),#15180,.F.);
#15453=ADVANCED_FACE('',(#2143),#15181,.F.);
#15454=ADVANCED_FACE('',(#2144),#15182,.F.);
#15455=ADVANCED_FACE('',(#2145),#15183,.F.);
#15456=ADVANCED_FACE('',(#2146),#15184,.F.);
#15457=ADVANCED_FACE('',(#2147),#15185,.F.);
#15458=ADVANCED_FACE('',(#2148),#15186,.F.);
#15459=ADVANCED_FACE('',(#2149),#15187,.F.);
#15460=ADVANCED_FACE('',(#2150),#15188,.F.);
#15461=ADVANCED_FACE('',(#2151),#15189,.F.);
#15462=ADVANCED_FACE('',(#2152),#15190,.F.);
#15463=ADVANCED_FACE('',(#2153),#15191,.F.);
#15464=ADVANCED_FACE('',(#2154),#15192,.F.);
#15465=ADVANCED_FACE('',(#2155),#15193,.F.);
#15466=ADVANCED_FACE('',(#2156),#15194,.F.);
#15467=ADVANCED_FACE('',(#2157,#1348,#1349,#1350),#1639,.T.);
#15468=ADVANCED_FACE('',(#2158),#1640,.F.);
#15469=ADVANCED_FACE('',(#2159,#1351,#1352,#1353,#1354,#1355,#1356,#1357,
#1358,#1359,#1360,#1361,#1362,#1363,#1364,#1365,#1366,#1367,#1368,#1369,
#1370,#1371,#1372),#1641,.T.);
#15470=ADVANCED_FACE('',(#2160),#1642,.T.);
#15471=ADVANCED_FACE('',(#2161,#1373,#1374,#1375,#1376,#1377,#1378,#1379,
#1380,#1381,#1382,#1383,#1384,#1385,#1386,#1387,#1388,#1389,#1390,#1391,
#1392,#1393,#1394),#1643,.T.);
#15472=ADVANCED_FACE('',(#2162),#1644,.T.);
#15473=ADVANCED_FACE('',(#2163),#1645,.T.);
#15474=ADVANCED_FACE('',(#2164,#1395,#1396,#1397),#1646,.F.);
#16370=CLOSED_SHELL('',(#15442,#15443,#15444,#15445,#15446,#15447,#15448,
#15449,#15450,#15451,#15452,#15453,#15454,#15455,#15456,#15457,#15458,#15459,
#15460,#15461,#15462,#15463,#15464,#15465,#15466,#15467,#15468,#15469,#15470,
#15471,#15472,#15473,#15474));
#17176=AXIS2_PLACEMENT_3D('',#23356,#18882,#18883);
#17177=AXIS2_PLACEMENT_3D('',#23357,#18884,#18885);
#17178=AXIS2_PLACEMENT_3D('',#23359,#18886,#18887);
#17179=AXIS2_PLACEMENT_3D('',#23362,#18889,#18890);
#17180=AXIS2_PLACEMENT_3D('',#23363,#18891,#18892);
#17181=AXIS2_PLACEMENT_3D('',#23365,#18893,#18894);
#17182=AXIS2_PLACEMENT_3D('',#23368,#18896,#18897);
#17183=AXIS2_PLACEMENT_3D('',#23369,#18898,#18899);
#17184=AXIS2_PLACEMENT_3D('',#23371,#18900,#18901);
#17185=AXIS2_PLACEMENT_3D('',#23374,#18903,#18904);
#17186=AXIS2_PLACEMENT_3D('',#23375,#18905,#18906);
#17187=AXIS2_PLACEMENT_3D('',#23377,#18907,#18908);
#17188=AXIS2_PLACEMENT_3D('',#23380,#18910,#18911);
#17189=AXIS2_PLACEMENT_3D('',#23381,#18912,#18913);
#17190=AXIS2_PLACEMENT_3D('',#23383,#18914,#18915);
#17191=AXIS2_PLACEMENT_3D('',#23386,#18917,#18918);
#17192=AXIS2_PLACEMENT_3D('',#23387,#18919,#18920);
#17193=AXIS2_PLACEMENT_3D('',#23389,#18921,#18922);
#17194=AXIS2_PLACEMENT_3D('',#23392,#18924,#18925);
#17195=AXIS2_PLACEMENT_3D('',#23393,#18926,#18927);
#17196=AXIS2_PLACEMENT_3D('',#23395,#18928,#18929);
#17197=AXIS2_PLACEMENT_3D('',#23398,#18931,#18932);
#17198=AXIS2_PLACEMENT_3D('',#23399,#18933,#18934);
#17199=AXIS2_PLACEMENT_3D('',#23401,#18935,#18936);
#17200=AXIS2_PLACEMENT_3D('',#23404,#18938,#18939);
#17201=AXIS2_PLACEMENT_3D('',#23405,#18940,#18941);
#17202=AXIS2_PLACEMENT_3D('',#23407,#18942,#18943);
#17203=AXIS2_PLACEMENT_3D('',#23410,#18945,#18946);
#17204=AXIS2_PLACEMENT_3D('',#23411,#18947,#18948);
#17205=AXIS2_PLACEMENT_3D('',#23413,#18949,#18950);
#17206=AXIS2_PLACEMENT_3D('',#23416,#18952,#18953);
#17207=AXIS2_PLACEMENT_3D('',#23417,#18954,#18955);
#17208=AXIS2_PLACEMENT_3D('',#23419,#18956,#18957);
#17209=AXIS2_PLACEMENT_3D('',#23422,#18959,#18960);
#17210=AXIS2_PLACEMENT_3D('',#23423,#18961,#18962);
#17211=AXIS2_PLACEMENT_3D('',#23425,#18963,#18964);
#17212=AXIS2_PLACEMENT_3D('',#23428,#18966,#18967);
#17213=AXIS2_PLACEMENT_3D('',#23429,#18968,#18969);
#17214=AXIS2_PLACEMENT_3D('',#23431,#18970,#18971);
#17215=AXIS2_PLACEMENT_3D('',#23434,#18973,#18974);
#17216=AXIS2_PLACEMENT_3D('',#23435,#18975,#18976);
#17217=AXIS2_PLACEMENT_3D('',#23437,#18977,#18978);
#17218=AXIS2_PLACEMENT_3D('',#23440,#18980,#18981);
#17219=AXIS2_PLACEMENT_3D('',#23441,#18982,#18983);
#17220=AXIS2_PLACEMENT_3D('',#23443,#18984,#18985);
#17221=AXIS2_PLACEMENT_3D('',#23446,#18987,#18988);
#17222=AXIS2_PLACEMENT_3D('',#23447,#18989,#18990);
#17223=AXIS2_PLACEMENT_3D('',#23449,#18991,#18992);
#17224=AXIS2_PLACEMENT_3D('',#23452,#18994,#18995);
#17225=AXIS2_PLACEMENT_3D('',#23453,#18996,#18997);
#17226=AXIS2_PLACEMENT_3D('',#23455,#18998,#18999);
#17227=AXIS2_PLACEMENT_3D('',#23458,#19001,#19002);
#17228=AXIS2_PLACEMENT_3D('',#23459,#19003,#19004);
#17229=AXIS2_PLACEMENT_3D('',#23461,#19005,#19006);
#17230=AXIS2_PLACEMENT_3D('',#23464,#19008,#19009);
#17231=AXIS2_PLACEMENT_3D('',#23465,#19010,#19011);
#17232=AXIS2_PLACEMENT_3D('',#23467,#19012,#19013);
#17233=AXIS2_PLACEMENT_3D('',#23470,#19015,#19016);
#17234=AXIS2_PLACEMENT_3D('',#23471,#19017,#19018);
#17235=AXIS2_PLACEMENT_3D('',#23473,#19019,#19020);
#17236=AXIS2_PLACEMENT_3D('',#23476,#19022,#19023);
#17237=AXIS2_PLACEMENT_3D('',#23477,#19024,#19025);
#17238=AXIS2_PLACEMENT_3D('',#23479,#19026,#19027);
#17239=AXIS2_PLACEMENT_3D('',#23482,#19029,#19030);
#17240=AXIS2_PLACEMENT_3D('',#23483,#19031,#19032);
#17241=AXIS2_PLACEMENT_3D('',#23485,#19033,#19034);
#17242=AXIS2_PLACEMENT_3D('',#23488,#19036,#19037);
#17243=AXIS2_PLACEMENT_3D('',#23489,#19038,#19039);
#17244=AXIS2_PLACEMENT_3D('',#23491,#19040,#19041);
#17245=AXIS2_PLACEMENT_3D('',#23494,#19043,#19044);
#17246=AXIS2_PLACEMENT_3D('',#23495,#19045,#19046);
#17247=AXIS2_PLACEMENT_3D('',#23497,#19047,#19048);
#17248=AXIS2_PLACEMENT_3D('',#23500,#19050,#19051);
#17249=AXIS2_PLACEMENT_3D('',#23501,#19052,#19053);
#17250=AXIS2_PLACEMENT_3D('',#23503,#19054,#19055);
#17251=AXIS2_PLACEMENT_3D('',#23506,#19057,#19058);
#17252=AXIS2_PLACEMENT_3D('',#23507,#19059,#19060);
#17253=AXIS2_PLACEMENT_3D('',#23516,#19065,#19066);
#17254=AXIS2_PLACEMENT_3D('',#23522,#19070,#19071);
#17255=AXIS2_PLACEMENT_3D('',#23531,#19076,#19077);
#17256=AXIS2_PLACEMENT_3D('',#23536,#19081,#19082);
#17257=AXIS2_PLACEMENT_3D('',#23540,#19085,#19086);
#17258=AXIS2_PLACEMENT_3D('',#23543,#19089,#19090);
#17259=AXIS2_PLACEMENT_3D('',#23544,#19091,#19092);
#18882=DIRECTION('axis',(0.,0.,1.));
#18883=DIRECTION('refdir',(1.,0.,0.));
#18884=DIRECTION('center_axis',(0.,1.,0.));
#18885=DIRECTION('ref_axis',(1.,0.,0.));
#18886=DIRECTION('center_axis',(0.,1.,0.));
#18887=DIRECTION('ref_axis',(1.,0.,0.));
#18888=DIRECTION('',(0.,1.,0.));
#18889=DIRECTION('center_axis',(0.,-1.,0.));
#18890=DIRECTION('ref_axis',(1.,0.,0.));
#18891=DIRECTION('center_axis',(0.,1.,0.));
#18892=DIRECTION('ref_axis',(1.,0.,0.));
#18893=DIRECTION('center_axis',(0.,1.,0.));
#18894=DIRECTION('ref_axis',(1.,0.,0.));
#18895=DIRECTION('',(0.,1.,0.));
#18896=DIRECTION('center_axis',(0.,-1.,0.));
#18897=DIRECTION('ref_axis',(1.,0.,0.));
#18898=DIRECTION('center_axis',(0.,1.,0.));
#18899=DIRECTION('ref_axis',(1.,0.,0.));
#18900=DIRECTION('center_axis',(0.,1.,0.));
#18901=DIRECTION('ref_axis',(1.,0.,0.));
#18902=DIRECTION('',(0.,1.,0.));
#18903=DIRECTION('center_axis',(0.,-1.,0.));
#18904=DIRECTION('ref_axis',(1.,0.,0.));
#18905=DIRECTION('center_axis',(0.,1.,0.));
#18906=DIRECTION('ref_axis',(1.,0.,0.));
#18907=DIRECTION('center_axis',(0.,1.,0.));
#18908=DIRECTION('ref_axis',(1.,0.,0.));
#18909=DIRECTION('',(0.,1.,0.));
#18910=DIRECTION('center_axis',(0.,-1.,0.));
#18911=DIRECTION('ref_axis',(1.,0.,0.));
#18912=DIRECTION('center_axis',(0.,1.,0.));
#18913=DIRECTION('ref_axis',(1.,0.,0.));
#18914=DIRECTION('center_axis',(0.,1.,0.));
#18915=DIRECTION('ref_axis',(1.,0.,0.));
#18916=DIRECTION('',(0.,1.,0.));
#18917=DIRECTION('center_axis',(0.,-1.,0.));
#18918=DIRECTION('ref_axis',(1.,0.,0.));
#18919=DIRECTION('center_axis',(0.,1.,0.));
#18920=DIRECTION('ref_axis',(1.,0.,0.));
#18921=DIRECTION('center_axis',(0.,1.,0.));
#18922=DIRECTION('ref_axis',(1.,0.,0.));
#18923=DIRECTION('',(0.,1.,0.));
#18924=DIRECTION('center_axis',(0.,-1.,0.));
#18925=DIRECTION('ref_axis',(1.,0.,0.));
#18926=DIRECTION('center_axis',(0.,1.,0.));
#18927=DIRECTION('ref_axis',(1.,0.,0.));
#18928=DIRECTION('center_axis',(0.,1.,0.));
#18929=DIRECTION('ref_axis',(1.,0.,0.));
#18930=DIRECTION('',(0.,1.,0.));
#18931=DIRECTION('center_axis',(0.,-1.,0.));
#18932=DIRECTION('ref_axis',(1.,0.,0.));
#18933=DIRECTION('center_axis',(0.,1.,0.));
#18934=DIRECTION('ref_axis',(1.,0.,0.));
#18935=DIRECTION('center_axis',(0.,1.,0.));
#18936=DIRECTION('ref_axis',(1.,0.,0.));
#18937=DIRECTION('',(0.,1.,0.));
#18938=DIRECTION('center_axis',(0.,-1.,0.));
#18939=DIRECTION('ref_axis',(1.,0.,0.));
#18940=DIRECTION('center_axis',(0.,1.,0.));
#18941=DIRECTION('ref_axis',(1.,0.,0.));
#18942=DIRECTION('center_axis',(0.,1.,0.));
#18943=DIRECTION('ref_axis',(1.,0.,0.));
#18944=DIRECTION('',(0.,1.,0.));
#18945=DIRECTION('center_axis',(0.,-1.,0.));
#18946=DIRECTION('ref_axis',(1.,0.,0.));
#18947=DIRECTION('center_axis',(0.,1.,0.));
#18948=DIRECTION('ref_axis',(1.,0.,0.));
#18949=DIRECTION('center_axis',(0.,1.,0.));
#18950=DIRECTION('ref_axis',(1.,0.,0.));
#18951=DIRECTION('',(0.,1.,0.));
#18952=DIRECTION('center_axis',(0.,-1.,0.));
#18953=DIRECTION('ref_axis',(1.,0.,0.));
#18954=DIRECTION('center_axis',(0.,1.,0.));
#18955=DIRECTION('ref_axis',(1.,0.,0.));
#18956=DIRECTION('center_axis',(0.,1.,0.));
#18957=DIRECTION('ref_axis',(1.,0.,0.));
#18958=DIRECTION('',(0.,1.,0.));
#18959=DIRECTION('center_axis',(0.,-1.,0.));
#18960=DIRECTION('ref_axis',(1.,0.,0.));
#18961=DIRECTION('center_axis',(0.,1.,0.));
#18962=DIRECTION('ref_axis',(1.,0.,0.));
#18963=DIRECTION('center_axis',(0.,1.,0.));
#18964=DIRECTION('ref_axis',(1.,0.,0.));
#18965=DIRECTION('',(0.,1.,0.));
#18966=DIRECTION('center_axis',(0.,-1.,0.));
#18967=DIRECTION('ref_axis',(1.,0.,0.));
#18968=DIRECTION('center_axis',(0.,1.,0.));
#18969=DIRECTION('ref_axis',(1.,0.,0.));
#18970=DIRECTION('center_axis',(0.,1.,0.));
#18971=DIRECTION('ref_axis',(1.,0.,0.));
#18972=DIRECTION('',(0.,1.,0.));
#18973=DIRECTION('center_axis',(0.,-1.,0.));
#18974=DIRECTION('ref_axis',(1.,0.,0.));
#18975=DIRECTION('center_axis',(0.,1.,0.));
#18976=DIRECTION('ref_axis',(1.,0.,0.));
#18977=DIRECTION('center_axis',(0.,1.,0.));
#18978=DIRECTION('ref_axis',(1.,0.,0.));
#18979=DIRECTION('',(0.,1.,0.));
#18980=DIRECTION('center_axis',(0.,-1.,0.));
#18981=DIRECTION('ref_axis',(1.,0.,0.));
#18982=DIRECTION('center_axis',(0.,1.,0.));
#18983=DIRECTION('ref_axis',(1.,0.,0.));
#18984=DIRECTION('center_axis',(0.,1.,0.));
#18985=DIRECTION('ref_axis',(1.,0.,0.));
#18986=DIRECTION('',(0.,1.,0.));
#18987=DIRECTION('center_axis',(0.,-1.,0.));
#18988=DIRECTION('ref_axis',(1.,0.,0.));
#18989=DIRECTION('center_axis',(0.,1.,0.));
#18990=DIRECTION('ref_axis',(1.,0.,0.));
#18991=DIRECTION('center_axis',(0.,1.,0.));
#18992=DIRECTION('ref_axis',(1.,0.,0.));
#18993=DIRECTION('',(0.,1.,0.));
#18994=DIRECTION('center_axis',(0.,-1.,0.));
#18995=DIRECTION('ref_axis',(1.,0.,0.));
#18996=DIRECTION('center_axis',(0.,1.,0.));
#18997=DIRECTION('ref_axis',(1.,0.,0.));
#18998=DIRECTION('center_axis',(0.,1.,0.));
#18999=DIRECTION('ref_axis',(1.,0.,0.));
#19000=DIRECTION('',(0.,1.,0.));
#19001=DIRECTION('center_axis',(0.,-1.,0.));
#19002=DIRECTION('ref_axis',(1.,0.,0.));
#19003=DIRECTION('center_axis',(0.,1.,0.));
#19004=DIRECTION('ref_axis',(1.,0.,0.));
#19005=DIRECTION('center_axis',(0.,1.,0.));
#19006=DIRECTION('ref_axis',(1.,0.,0.));
#19007=DIRECTION('',(0.,1.,0.));
#19008=DIRECTION('center_axis',(0.,-1.,0.));
#19009=DIRECTION('ref_axis',(1.,0.,0.));
#19010=DIRECTION('center_axis',(0.,1.,0.));
#19011=DIRECTION('ref_axis',(1.,0.,0.));
#19012=DIRECTION('center_axis',(0.,1.,0.));
#19013=DIRECTION('ref_axis',(1.,0.,0.));
#19014=DIRECTION('',(0.,1.,0.));
#19015=DIRECTION('center_axis',(0.,-1.,0.));
#19016=DIRECTION('ref_axis',(1.,0.,0.));
#19017=DIRECTION('center_axis',(0.,1.,0.));
#19018=DIRECTION('ref_axis',(1.,0.,0.));
#19019=DIRECTION('center_axis',(0.,1.,0.));
#19020=DIRECTION('ref_axis',(1.,0.,0.));
#19021=DIRECTION('',(0.,1.,0.));
#19022=DIRECTION('center_axis',(0.,-1.,0.));
#19023=DIRECTION('ref_axis',(1.,0.,0.));
#19024=DIRECTION('center_axis',(0.,1.,0.));
#19025=DIRECTION('ref_axis',(1.,0.,0.));
#19026=DIRECTION('center_axis',(0.,1.,0.));
#19027=DIRECTION('ref_axis',(1.,0.,0.));
#19028=DIRECTION('',(0.,1.,0.));
#19029=DIRECTION('center_axis',(0.,-1.,0.));
#19030=DIRECTION('ref_axis',(1.,0.,0.));
#19031=DIRECTION('center_axis',(0.,1.,0.));
#19032=DIRECTION('ref_axis',(1.,0.,0.));
#19033=DIRECTION('center_axis',(0.,1.,0.));
#19034=DIRECTION('ref_axis',(1.,0.,0.));
#19035=DIRECTION('',(0.,1.,0.));
#19036=DIRECTION('center_axis',(0.,-1.,0.));
#19037=DIRECTION('ref_axis',(1.,0.,0.));
#19038=DIRECTION('center_axis',(0.,0.,1.));
#19039=DIRECTION('ref_axis',(1.,0.,0.));
#19040=DIRECTION('center_axis',(0.,0.,1.));
#19041=DIRECTION('ref_axis',(1.,0.,0.));
#19042=DIRECTION('',(0.,0.,1.));
#19043=DIRECTION('center_axis',(0.,0.,-1.));
#19044=DIRECTION('ref_axis',(1.,0.,0.));
#19045=DIRECTION('center_axis',(0.,0.,1.));
#19046=DIRECTION('ref_axis',(1.,0.,0.));
#19047=DIRECTION('center_axis',(0.,0.,1.));
#19048=DIRECTION('ref_axis',(1.,0.,0.));
#19049=DIRECTION('',(0.,0.,1.));
#19050=DIRECTION('center_axis',(0.,0.,-1.));
#19051=DIRECTION('ref_axis',(1.,0.,0.));
#19052=DIRECTION('center_axis',(0.,0.,1.));
#19053=DIRECTION('ref_axis',(1.,0.,0.));
#19054=DIRECTION('center_axis',(0.,0.,1.));
#19055=DIRECTION('ref_axis',(1.,0.,0.));
#19056=DIRECTION('',(0.,0.,1.));
#19057=DIRECTION('center_axis',(0.,0.,-1.));
#19058=DIRECTION('ref_axis',(1.,0.,0.));
#19059=DIRECTION('center_axis',(0.,0.,1.));
#19060=DIRECTION('ref_axis',(1.,0.,0.));
#19061=DIRECTION('',(-1.,0.,0.));
#19062=DIRECTION('',(0.,1.,0.));
#19063=DIRECTION('',(1.,0.,0.));
#19064=DIRECTION('',(0.,1.,0.));
#19065=DIRECTION('center_axis',(0.,1.,0.));
#19066=DIRECTION('ref_axis',(1.,0.,0.));
#19067=DIRECTION('',(0.,0.,-1.));
#19068=DIRECTION('',(1.,0.,0.));
#19069=DIRECTION('',(0.,0.,1.));
#19070=DIRECTION('center_axis',(0.,1.,0.));
#19071=DIRECTION('ref_axis',(-1.,0.,0.));
#19072=DIRECTION('',(-1.,0.,0.));
#19073=DIRECTION('',(0.,0.,1.));
#19074=DIRECTION('',(-1.,0.,0.));
#19075=DIRECTION('',(0.,0.,1.));
#19076=DIRECTION('center_axis',(1.,0.,0.));
#19077=DIRECTION('ref_axis',(0.,1.,0.));
#19078=DIRECTION('',(0.,1.,0.));
#19079=DIRECTION('',(0.,1.,0.));
#19080=DIRECTION('',(0.,0.,1.));
#19081=DIRECTION('center_axis',(0.,-1.,0.));
#19082=DIRECTION('ref_axis',(1.,0.,0.));
#19083=DIRECTION('',(1.,0.,0.));
#19084=DIRECTION('',(0.,0.,1.));
#19085=DIRECTION('center_axis',(-1.,0.,0.));
#19086=DIRECTION('ref_axis',(0.,-1.,0.));
#19087=DIRECTION('',(0.,-1.,0.));
#19088=DIRECTION('',(0.,-1.,0.));
#19089=DIRECTION('center_axis',(0.,0.,1.));
#19090=DIRECTION('ref_axis',(1.,0.,0.));
#19091=DIRECTION('center_axis',(0.,0.,1.));
#19092=DIRECTION('ref_axis',(1.,0.,0.));
#23356=CARTESIAN_POINT('',(0.,0.,0.));
#23357=CARTESIAN_POINT('Origin',(23.,-2.5,14.));
#23358=CARTESIAN_POINT('',(22.775,-2.4,14.));
#23359=CARTESIAN_POINT('Origin',(23.,-2.4,14.));
#23360=CARTESIAN_POINT('',(22.775,-0.6,14.));
#23361=CARTESIAN_POINT('',(22.775,-2.5,14.));
#23362=CARTESIAN_POINT('Origin',(23.,-0.6,14.));
#23363=CARTESIAN_POINT('Origin',(23.,-2.5,4.));
#23364=CARTESIAN_POINT('',(22.775,-2.4,4.));
#23365=CARTESIAN_POINT('Origin',(23.,-2.4,4.));
#23366=CARTESIAN_POINT('',(22.775,-0.6,4.));
#23367=CARTESIAN_POINT('',(22.775,-2.5,4.));
#23368=CARTESIAN_POINT('Origin',(23.,-0.6,4.));
#23369=CARTESIAN_POINT('Origin',(16.161522368915,-2.5,7.16152236891498));
#23370=CARTESIAN_POINT('',(15.996522368915,-2.4,7.16152236891498));
#23371=CARTESIAN_POINT('Origin',(16.161522368915,-2.4,7.16152236891498));
#23372=CARTESIAN_POINT('',(15.996522368915,-0.6,7.16152236891498));
#23373=CARTESIAN_POINT('',(15.996522368915,-2.5,7.16152236891498));
#23374=CARTESIAN_POINT('Origin',(16.161522368915,-0.6,7.16152236891498));
#23375=CARTESIAN_POINT('Origin',(16.161522368915,-2.5,10.838477631085));
#23376=CARTESIAN_POINT('',(15.996522368915,-2.4,10.838477631085));
#23377=CARTESIAN_POINT('Origin',(16.161522368915,-2.4,10.838477631085));
#23378=CARTESIAN_POINT('',(15.996522368915,-0.6,10.838477631085));
#23379=CARTESIAN_POINT('',(15.996522368915,-2.5,10.838477631085));
#23380=CARTESIAN_POINT('Origin',(16.161522368915,-0.6,10.838477631085));
#23381=CARTESIAN_POINT('Origin',(19.838477631085,-2.5,10.838477631085));
#23382=CARTESIAN_POINT('',(19.673477631085,-2.4,10.838477631085));
#23383=CARTESIAN_POINT('Origin',(19.838477631085,-2.4,10.838477631085));
#23384=CARTESIAN_POINT('',(19.673477631085,-0.6,10.838477631085));
#23385=CARTESIAN_POINT('',(19.673477631085,-2.5,10.838477631085));
#23386=CARTESIAN_POINT('Origin',(19.838477631085,-0.6,10.838477631085));
#23387=CARTESIAN_POINT('Origin',(19.838477631085,-2.5,7.16152236891498));
#23388=CARTESIAN_POINT('',(19.673477631085,-2.4,7.16152236891498));
#23389=CARTESIAN_POINT('Origin',(19.838477631085,-2.4,7.16152236891498));
#23390=CARTESIAN_POINT('',(19.673477631085,-0.6,7.16152236891498));
#23391=CARTESIAN_POINT('',(19.673477631085,-2.5,7.16152236891498));
#23392=CARTESIAN_POINT('Origin',(19.838477631085,-0.6,7.16152236891498));
#23393=CARTESIAN_POINT('Origin',(18.,-2.5,9.));
#23394=CARTESIAN_POINT('',(15.65,-2.4,9.));
#23395=CARTESIAN_POINT('Origin',(18.,-2.4,9.));
#23396=CARTESIAN_POINT('',(15.65,-0.6,9.));
#23397=CARTESIAN_POINT('',(15.65,-2.5,9.));
#23398=CARTESIAN_POINT('Origin',(18.,-0.6,9.));
#23399=CARTESIAN_POINT('Origin',(10.5150757595082,-2.5,7.51507575950825));
#23400=CARTESIAN_POINT('',(10.3500757595083,-2.4,7.51507575950825));
#23401=CARTESIAN_POINT('Origin',(10.5150757595082,-2.4,7.51507575950825));
#23402=CARTESIAN_POINT('',(10.3500757595083,-0.6,7.51507575950825));
#23403=CARTESIAN_POINT('',(10.3500757595083,-2.5,7.51507575950825));
#23404=CARTESIAN_POINT('Origin',(10.5150757595082,-0.6,7.51507575950825));
#23405=CARTESIAN_POINT('Origin',(10.5150757595082,-2.5,10.4849242404918));
#23406=CARTESIAN_POINT('',(10.3500757595083,-2.4,10.4849242404918));
#23407=CARTESIAN_POINT('Origin',(10.5150757595082,-2.4,10.4849242404918));
#23408=CARTESIAN_POINT('',(10.3500757595083,-0.6,10.4849242404918));
#23409=CARTESIAN_POINT('',(10.3500757595083,-2.5,10.4849242404918));
#23410=CARTESIAN_POINT('Origin',(10.5150757595082,-0.6,10.4849242404918));
#23411=CARTESIAN_POINT('Origin',(13.4849242404918,-2.5,10.4849242404918));
#23412=CARTESIAN_POINT('',(13.3199242404918,-2.4,10.4849242404918));
#23413=CARTESIAN_POINT('Origin',(13.4849242404918,-2.4,10.4849242404918));
#23414=CARTESIAN_POINT('',(13.3199242404918,-0.6,10.4849242404918));
#23415=CARTESIAN_POINT('',(13.3199242404918,-2.5,10.4849242404918));
#23416=CARTESIAN_POINT('Origin',(13.4849242404918,-0.6,10.4849242404918));
#23417=CARTESIAN_POINT('Origin',(13.4849242404918,-2.5,7.51507575950825));
#23418=CARTESIAN_POINT('',(13.3199242404918,-2.4,7.51507575950825));
#23419=CARTESIAN_POINT('Origin',(13.4849242404918,-2.4,7.51507575950825));
#23420=CARTESIAN_POINT('',(13.3199242404918,-0.6,7.51507575950825));
#23421=CARTESIAN_POINT('',(13.3199242404918,-2.5,7.51507575950825));
#23422=CARTESIAN_POINT('Origin',(13.4849242404918,-0.6,7.51507575950825));
#23423=CARTESIAN_POINT('Origin',(12.,-2.5,9.));
#23424=CARTESIAN_POINT('',(10.4,-2.4,9.));
#23425=CARTESIAN_POINT('Origin',(12.,-2.4,9.));
#23426=CARTESIAN_POINT('',(10.4,-0.6,9.));
#23427=CARTESIAN_POINT('',(10.4,-2.5,9.));
#23428=CARTESIAN_POINT('Origin',(12.,-0.6,9.));
#23429=CARTESIAN_POINT('Origin',(4.16152236891498,-2.5,7.16152236891498));
#23430=CARTESIAN_POINT('',(3.99652236891498,-2.4,7.16152236891498));
#23431=CARTESIAN_POINT('Origin',(4.16152236891498,-2.4,7.16152236891498));
#23432=CARTESIAN_POINT('',(3.99652236891498,-0.6,7.16152236891498));
#23433=CARTESIAN_POINT('',(3.99652236891498,-2.5,7.16152236891498));
#23434=CARTESIAN_POINT('Origin',(4.16152236891498,-0.6,7.16152236891498));
#23435=CARTESIAN_POINT('Origin',(4.16152236891498,-2.5,10.838477631085));
#23436=CARTESIAN_POINT('',(3.99652236891498,-2.4,10.838477631085));
#23437=CARTESIAN_POINT('Origin',(4.16152236891498,-2.4,10.838477631085));
#23438=CARTESIAN_POINT('',(3.99652236891498,-0.6,10.838477631085));
#23439=CARTESIAN_POINT('',(3.99652236891498,-2.5,10.838477631085));
#23440=CARTESIAN_POINT('Origin',(4.16152236891498,-0.6,10.838477631085));
#23441=CARTESIAN_POINT('Origin',(7.83847763108502,-2.5,10.838477631085));
#23442=CARTESIAN_POINT('',(7.67347763108502,-2.4,10.838477631085));
#23443=CARTESIAN_POINT('Origin',(7.83847763108502,-2.4,10.838477631085));
#23444=CARTESIAN_POINT('',(7.67347763108502,-0.6,10.838477631085));
#23445=CARTESIAN_POINT('',(7.67347763108502,-2.5,10.838477631085));
#23446=CARTESIAN_POINT('Origin',(7.83847763108502,-0.6,10.838477631085));
#23447=CARTESIAN_POINT('Origin',(7.83847763108502,-2.5,7.16152236891498));
#23448=CARTESIAN_POINT('',(7.67347763108502,-2.4,7.16152236891498));
#23449=CARTESIAN_POINT('Origin',(7.83847763108502,-2.4,7.16152236891498));
#23450=CARTESIAN_POINT('',(7.67347763108502,-0.6,7.16152236891498));
#23451=CARTESIAN_POINT('',(7.67347763108502,-2.5,7.16152236891498));
#23452=CARTESIAN_POINT('Origin',(7.83847763108502,-0.6,7.16152236891498));
#23453=CARTESIAN_POINT('Origin',(6.,-2.5,9.));
#23454=CARTESIAN_POINT('',(3.65,-2.4,9.));
#23455=CARTESIAN_POINT('Origin',(6.,-2.4,9.));
#23456=CARTESIAN_POINT('',(3.65,-0.6,9.));
#23457=CARTESIAN_POINT('',(3.65,-2.5,9.));
#23458=CARTESIAN_POINT('Origin',(6.,-0.6,9.));
#23459=CARTESIAN_POINT('Origin',(-1.48492424049175,-2.5,7.51507575950825));
#23460=CARTESIAN_POINT('',(-1.64992424049175,-2.4,7.51507575950825));
#23461=CARTESIAN_POINT('Origin',(-1.48492424049175,-2.4,7.51507575950825));
#23462=CARTESIAN_POINT('',(-1.64992424049175,-0.6,7.51507575950825));
#23463=CARTESIAN_POINT('',(-1.64992424049175,-2.5,7.51507575950825));
#23464=CARTESIAN_POINT('Origin',(-1.48492424049175,-0.6,7.51507575950825));
#23465=CARTESIAN_POINT('Origin',(-1.48492424049175,-2.5,10.4849242404918));
#23466=CARTESIAN_POINT('',(-1.64992424049175,-2.4,10.4849242404918));
#23467=CARTESIAN_POINT('Origin',(-1.48492424049175,-2.4,10.4849242404918));
#23468=CARTESIAN_POINT('',(-1.64992424049175,-0.6,10.4849242404918));
#23469=CARTESIAN_POINT('',(-1.64992424049175,-2.5,10.4849242404918));
#23470=CARTESIAN_POINT('Origin',(-1.48492424049175,-0.6,10.4849242404918));
#23471=CARTESIAN_POINT('Origin',(1.48492424049175,-2.5,10.4849242404918));
#23472=CARTESIAN_POINT('',(1.31992424049175,-2.4,10.4849242404918));
#23473=CARTESIAN_POINT('Origin',(1.48492424049175,-2.4,10.4849242404918));
#23474=CARTESIAN_POINT('',(1.31992424049175,-0.6,10.4849242404918));
#23475=CARTESIAN_POINT('',(1.31992424049175,-2.5,10.4849242404918));
#23476=CARTESIAN_POINT('Origin',(1.48492424049175,-0.6,10.4849242404918));
#23477=CARTESIAN_POINT('Origin',(1.48492424049175,-2.5,7.51507575950825));
#23478=CARTESIAN_POINT('',(1.31992424049175,-2.4,7.51507575950825));
#23479=CARTESIAN_POINT('Origin',(1.48492424049175,-2.4,7.51507575950825));
#23480=CARTESIAN_POINT('',(1.31992424049175,-0.6,7.51507575950825));
#23481=CARTESIAN_POINT('',(1.31992424049175,-2.5,7.51507575950825));
#23482=CARTESIAN_POINT('Origin',(1.48492424049175,-0.6,7.51507575950825));
#23483=CARTESIAN_POINT('Origin',(0.,-2.5,9.));
#23484=CARTESIAN_POINT('',(-1.6,-2.4,9.));
#23485=CARTESIAN_POINT('Origin',(0.,-2.4,9.));
#23486=CARTESIAN_POINT('',(-1.6,-0.6,9.));
#23487=CARTESIAN_POINT('',(-1.6,-2.5,9.));
#23488=CARTESIAN_POINT('Origin',(0.,-0.6,9.));
#23489=CARTESIAN_POINT('Origin',(-2.,-5.,0.9));
#23490=CARTESIAN_POINT('',(-2.33,-5.,1.));
#23491=CARTESIAN_POINT('Origin',(-2.,-5.,1.));
#23492=CARTESIAN_POINT('',(-2.33,-5.,2.));
#23493=CARTESIAN_POINT('',(-2.33,-5.,0.9));
#23494=CARTESIAN_POINT('Origin',(-2.,-5.,2.));
#23495=CARTESIAN_POINT('Origin',(9.,-5.,0.9));
#23496=CARTESIAN_POINT('',(8.67,-5.,1.));
#23497=CARTESIAN_POINT('Origin',(9.,-5.,1.));
#23498=CARTESIAN_POINT('',(8.67,-5.,2.));
#23499=CARTESIAN_POINT('',(8.67,-5.,0.9));
#23500=CARTESIAN_POINT('Origin',(9.,-5.,2.));
#23501=CARTESIAN_POINT('Origin',(22.,-5.,0.9));
#23502=CARTESIAN_POINT('',(21.67,-5.,1.));
#23503=CARTESIAN_POINT('Origin',(22.,-5.,1.));
#23504=CARTESIAN_POINT('',(21.67,-5.,2.));
#23505=CARTESIAN_POINT('',(21.67,-5.,0.9));
#23506=CARTESIAN_POINT('Origin',(22.,-5.,2.));
#23507=CARTESIAN_POINT('Origin',(-3.5,-6.,2.));
#23508=CARTESIAN_POINT('',(23.5,-6.,2.));
#23509=CARTESIAN_POINT('',(-3.5,-6.,2.));
#23510=CARTESIAN_POINT('',(23.5,-6.,2.));
#23511=CARTESIAN_POINT('',(23.5,-2.4,2.));
#23512=CARTESIAN_POINT('',(23.5,-6.,2.));
#23513=CARTESIAN_POINT('',(-3.5,-2.4,2.));
#23514=CARTESIAN_POINT('',(-3.5,-2.4,2.));
#23515=CARTESIAN_POINT('',(-3.5,-6.,2.));
#23516=CARTESIAN_POINT('Origin',(10.,-6.,1.5));
#23517=CARTESIAN_POINT('',(-3.5,-6.,1.));
#23518=CARTESIAN_POINT('',(-3.5,-6.,2.));
#23519=CARTESIAN_POINT('',(23.5,-6.,1.));
#23520=CARTESIAN_POINT('',(-3.5,-6.,1.));
#23521=CARTESIAN_POINT('',(23.5,-6.,1.));
#23522=CARTESIAN_POINT('Origin',(23.5,-0.6,1.));
#23523=CARTESIAN_POINT('',(23.5,-0.6,1.));
#23524=CARTESIAN_POINT('',(-3.5,-0.6,1.));
#23525=CARTESIAN_POINT('',(23.5,-0.6,1.));
#23526=CARTESIAN_POINT('',(-3.5,-0.6,16.));
#23527=CARTESIAN_POINT('',(-3.5,-0.6,1.));
#23528=CARTESIAN_POINT('',(23.5,-0.6,16.));
#23529=CARTESIAN_POINT('',(23.5,-0.6,16.));
#23530=CARTESIAN_POINT('',(23.5,-0.6,1.));
#23531=CARTESIAN_POINT('Origin',(23.5,-2.4,1.));
#23532=CARTESIAN_POINT('',(23.5,-6.,1.));
#23533=CARTESIAN_POINT('',(23.5,-2.4,16.));
#23534=CARTESIAN_POINT('',(23.5,-2.4,16.));
#23535=CARTESIAN_POINT('',(23.5,-2.4,1.));
#23536=CARTESIAN_POINT('Origin',(-3.5,-2.4,1.));
#23537=CARTESIAN_POINT('',(-3.5,-2.4,16.));
#23538=CARTESIAN_POINT('',(-3.5,-2.4,16.));
#23539=CARTESIAN_POINT('',(-3.5,-2.4,1.));
#23540=CARTESIAN_POINT('Origin',(-3.5,-0.6,1.));
#23541=CARTESIAN_POINT('',(-3.5,-0.6,1.));
#23542=CARTESIAN_POINT('',(-3.5,-0.6,16.));
#23543=CARTESIAN_POINT('Origin',(10.,-1.5,16.));
#23544=CARTESIAN_POINT('Origin',(10.,-1.5,1.));
#62614=UNCERTAINTY_MEASURE_WITH_UNIT(LENGTH_MEASURE(0.001),#62759,
'DISTANCE_ACCURACY_VALUE',
'Maximum model space distance between geometric entities at asserted c
onnectivities');
#62684=UNCERTAINTY_MEASURE_WITH_UNIT(LENGTH_MEASURE(0.001),#62759,
'DISTANCE_ACCURACY_VALUE',
'Maximum model space distance between geometric entities at asserted c
onnectivities');
#62688=(
GEOMETRIC_REPRESENTATION_CONTEXT(3)
GLOBAL_UNCERTAINTY_ASSIGNED_CONTEXT((#62614))
GLOBAL_UNIT_ASSIGNED_CONTEXT((#62759,#62761,#62762))
REPRESENTATION_CONTEXT('','3D')
);
#62758=(
GEOMETRIC_REPRESENTATION_CONTEXT(3)
GLOBAL_UNCERTAINTY_ASSIGNED_CONTEXT((#62684))
GLOBAL_UNIT_ASSIGNED_CONTEXT((#62759,#62761,#62762))
REPRESENTATION_CONTEXT('','3D')
);
#62759=(
LENGTH_UNIT()
NAMED_UNIT(*)
SI_UNIT(.CENTI.,.METRE.)
);
#62761=(
NAMED_UNIT(*)
PLANE_ANGLE_UNIT()
SI_UNIT($,.RADIAN.)
);
#62762=(
NAMED_UNIT(*)
SI_UNIT($,.STERADIAN.)
SOLID_ANGLE_UNIT()
);
#62766=SHAPE_DEFINITION_REPRESENTATION(#62839,#63034);
#62839=PRODUCT_DEFINITION_SHAPE('',$,#63108);
#63034=SHAPE_REPRESENTATION('',(#17176),#62688);
#63104=PRODUCT_DEFINITION_CONTEXT('part definition',#63325,'design');
#63108=PRODUCT_DEFINITION('Bearing plate','Bearing plate',#63181,#63104);
#63181=PRODUCT_DEFINITION_FORMATION('',$,#63330);
#63325=APPLICATION_CONTEXT(
'Core Data for Automotive Mechanical Design Process');
#63326=PRODUCT_CONTEXT('part definition',#63325,'mechanical');
#63330=PRODUCT('Bearing plate','Bearing plate','Bearing plate',(#63326));
#63456=COLOUR_RGB('Grey',0.48,0.52,0.57);
#63457=FILL_AREA_STYLE_COLOUR('',#63456);
#63458=FILL_AREA_STYLE('',(#63457));
#63459=SURFACE_STYLE_FILL_AREA(#63458);
#63460=SURFACE_SIDE_STYLE('',(#63459));
#63461=SURFACE_STYLE_USAGE(.BOTH.,#63460);
#63462=PRESENTATION_STYLE_ASSIGNMENT((#63461));
ENDSEC;
END-ISO-10303-21;
